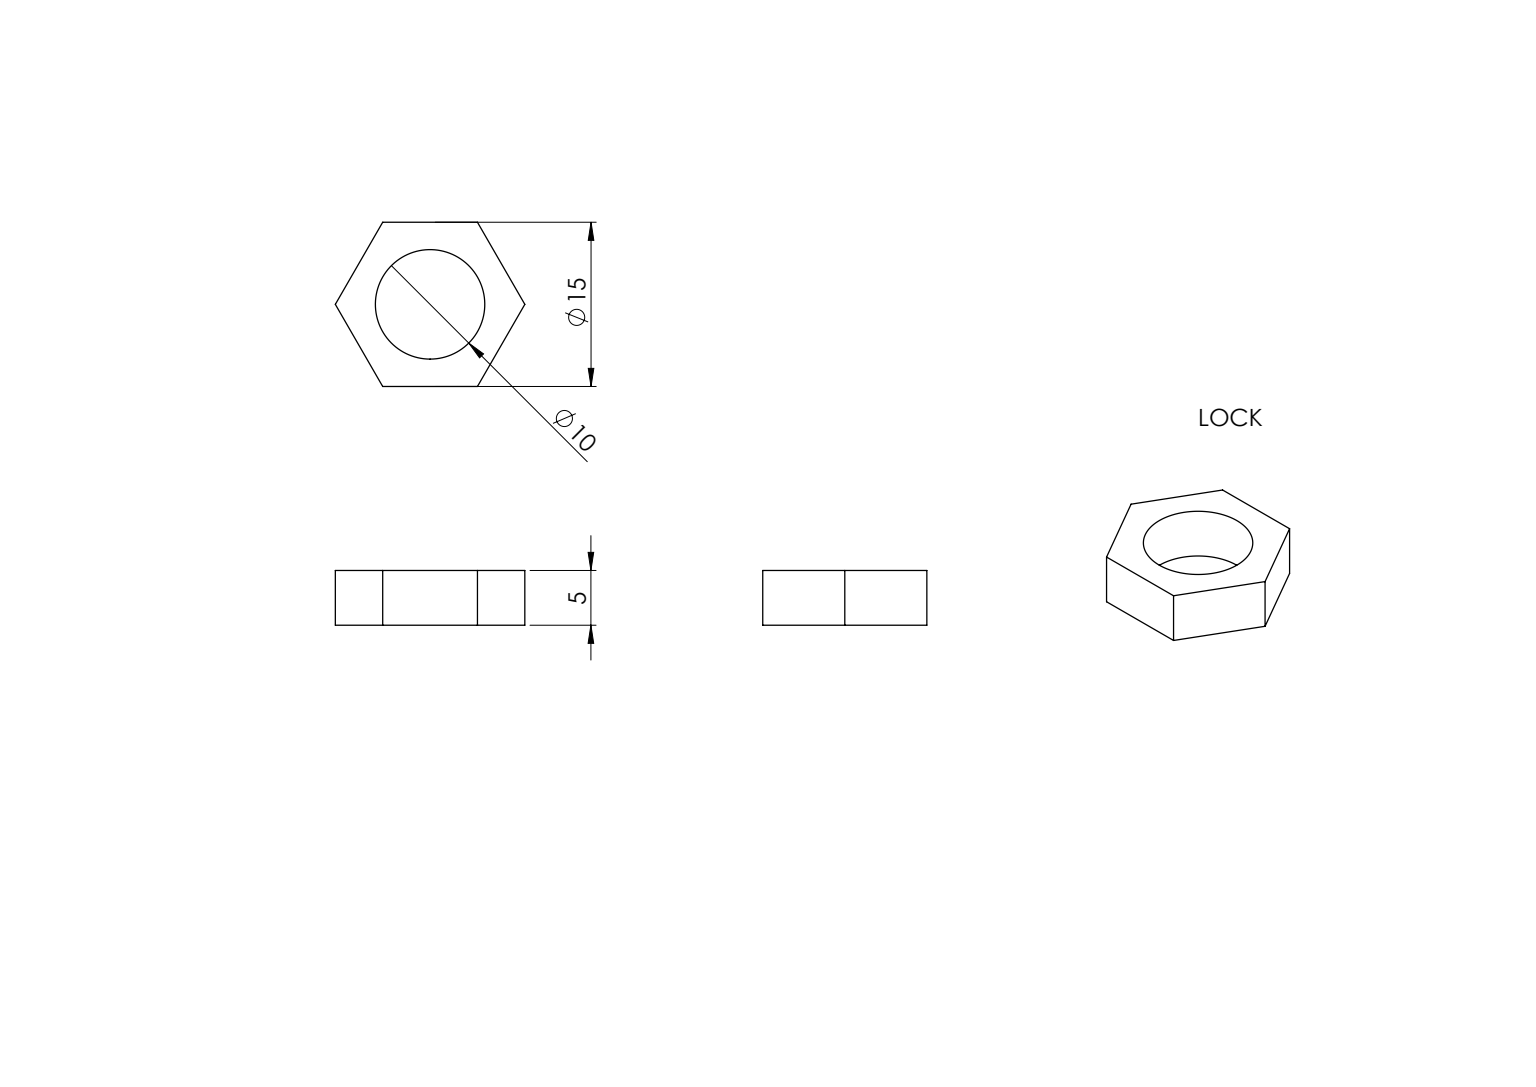
ISO-10303-21;
HEADER;
FILE_DESCRIPTION (('STEP AP214'),
    '1' );
FILE_NAME ('lock.step',
    '2026-10-27T14:18:53',
    ( '' ),
    ( '' ),
    'SwSTEP 2.0',
    'SolidWorks 2026',
    '' );
FILE_SCHEMA (( 'AUTOMOTIVE_DESIGN' ));
ENDSEC;

DATA;
#37=AXIS2_PLACEMENT_3D ( 'NONE', #854, #5957, #5527 ) ;
#40=MECHANICAL_DESIGN_GEOMETRIC_PRESENTATION_REPRESENTATION('',(#808),#5082);
#52=VERTEX_POINT ( 'NONE', #526 ) ;
#68=( NAMED_UNIT ( * ) SI_UNIT ( $, .STERADIAN. ) SOLID_ANGLE_UNIT ( ) );
#112=VECTOR ( 'NONE', #1206, 1000.000000000000000 ) ;
#117=EDGE_LOOP ( 'NONE', ( #4692, #1220, #1894, #1366 ) ) ;
#138=CYLINDRICAL_SURFACE ( 'NONE', #1374, 5.000000000000004441 ) ;
#157=UNCERTAINTY_MEASURE_WITH_UNIT (LENGTH_MEASURE( 1.000000000000000082E-05 ), #285, 'distance_accuracy_value', 'NONE');
#178=CARTESIAN_POINT ( 'NONE',  ( -53.66025403784439618, 45.00000000000000000, 45.00000000000001421 ) ) ;
#187=EDGE_LOOP ( 'NONE', ( #1142, #4922, #3638, #5470 ) ) ;
#212=CARTESIAN_POINT ( 'NONE',  ( -53.66025403784439618, 45.00000000000000000, 45.00000000000001421 ) ) ;
#225=VERTEX_POINT ( 'NONE', #2651 ) ;
#252=CARTESIAN_POINT ( 'NONE',  ( -53.66025403784439618, 40.00000000000000000, 45.00000000000001421 ) ) ;
#278=EDGE_CURVE ( 'NONE', #1461, #3435, #2305, .T. ) ;
#285=( LENGTH_UNIT ( ) NAMED_UNIT ( * ) SI_UNIT ( .MILLI., .METRE. ) );
#298=VECTOR ( 'NONE', #2052, 1000.000000000000227 ) ;
#301=EDGE_CURVE ( 'NONE', #4985, #4357, #4292, .T. ) ;
#309=DIRECTION ( 'NONE',  ( -0.000000000000000000, -1.000000000000000000, -0.000000000000000000 ) ) ;
#322=ORIENTED_EDGE ( 'NONE', *, *, #1089, .F. ) ;
#332=( GEOMETRIC_REPRESENTATION_CONTEXT ( 3 ) GLOBAL_UNCERTAINTY_ASSIGNED_CONTEXT ( ( #1483 ) ) GLOBAL_UNIT_ASSIGNED_CONTEXT ( ( #2789, #1481, #68 ) ) REPRESENTATION_CONTEXT ( 'NONE', 'WORKASPACE' ) );
#335=DIRECTION ( 'NONE',  ( -0.8660254037844390407, 0.000000000000000000, -0.4999999999999993894 ) ) ;
#348=FACE_BOUND ( 'NONE', #3880, .T. ) ;
#364=AXIS2_PLACEMENT_3D ( 'NONE', #2626, #335, #1690 ) ;
#378=CARTESIAN_POINT ( 'NONE',  ( -53.66025403784439618, 45.00000000000000000, 45.00000000000001421 ) ) ;
#394=STYLED_ITEM('',(#6013),#2189);
#396=EDGE_CURVE ( 'NONE', #4357, #4985, #5381, .T. ) ;
#434=CARTESIAN_POINT ( 'NONE',  ( -45.00000000000001421, 40.00000000000000000, 39.99999999999999289 ) ) ;
#465=ORIENTED_EDGE ( 'NONE', *, *, #3725, .F. ) ;
#483=SURFACE_STYLE_USAGE ( .BOTH. , #3752 ) ;
#514=EDGE_LOOP ( 'NONE', ( #4207, #2897 ) ) ;
#526=CARTESIAN_POINT ( 'NONE',  ( -40.66987298107781612, 40.00000000000000000, 37.50000000000000000 ) ) ;
#540=ADVANCED_FACE ( 'NONE', ( #2030 ), #4290, .F. ) ;
#542=VERTEX_POINT ( 'NONE', #968 ) ;
#560=CARTESIAN_POINT ( 'NONE',  ( -40.66987298107781612, 45.00000000000000000, 37.50000000000000000 ) ) ;
#571=( NAMED_UNIT ( * ) SI_UNIT ( $, .STERADIAN. ) SOLID_ANGLE_UNIT ( ) );
#585=ORIENTED_EDGE ( 'NONE', *, *, #2005, .F. ) ;
#588=DIRECTION ( 'NONE',  ( -0.000000000000000000, -1.000000000000000000, -0.000000000000000000 ) ) ;
#593=DIRECTION ( 'NONE',  ( 0.5000000000000004441, 0.000000000000000000, 0.8660254037844383745 ) ) ;
#637=UNCERTAINTY_MEASURE_WITH_UNIT (LENGTH_MEASURE( 1.000000000000000082E-05 ), #2820, 'distance_accuracy_value', 'NONE');
#642=EDGE_CURVE ( 'NONE', #3435, #4780, #1614, .T. ) ;
#643=ADVANCED_FACE ( 'NONE', ( #3491, #4470 ), #669, .F. ) ;
#656=EDGE_CURVE ( 'NONE', #3756, #3717, #1676, .T. ) ;
#667=DIRECTION ( 'NONE',  ( 1.000000000000000000, 0.000000000000000000, 0.000000000000000000 ) ) ;
#669=PLANE ( 'NONE',  #4650 ) ;
#700=PRODUCT_DEFINITION_CONTEXT ( 'detailed design', #4605, 'design' ) ;
#722=DIRECTION ( 'NONE',  ( 0.8660254037844383745, 0.000000000000000000, -0.5000000000000004441 ) ) ;
#754=LINE ( 'NONE', #5791, #1297 ) ;
#798=ORIENTED_EDGE ( 'NONE', *, *, #4836, .F. ) ;
#808=STYLED_ITEM ( 'NONE', ( #3256 ), #3558 ) ;
#820=CARTESIAN_POINT ( 'NONE',  ( -40.66987298107780902, 45.00000000000000000, 52.49999999999999289 ) ) ;
#854=CARTESIAN_POINT ( 'NONE',  ( -45.00000000000001421, 40.00000000000000000, 45.00000000000000000 ) ) ;
#894=DIRECTION ( 'NONE',  ( -0.000000000000000000, -1.000000000000000000, -0.000000000000000000 ) ) ;
#900=VECTOR ( 'NONE', #3820, 1000.000000000000000 ) ;
#909=PRODUCT_DEFINITION_FORMATION_WITH_SPECIFIED_SOURCE ( 'ANY', '', #5230, .NOT_KNOWN. ) ;
#922=ORIENTED_EDGE ( 'NONE', *, *, #1895, .T. ) ;
#968=CARTESIAN_POINT ( 'NONE',  ( -49.33012701892221230, 45.00000000000000000, 37.50000000000000000 ) ) ;
#979=ORIENTED_EDGE ( 'NONE', *, *, #5237, .F. ) ;
#985=DIRECTION ( 'NONE',  ( -0.000000000000000000, -1.000000000000000000, -0.000000000000000000 ) ) ;
#1001=SURFACE_STYLE_FILL_AREA ( #1903 ) ;
#1006=DIRECTION ( 'NONE',  ( 0.000000000000000000, 0.000000000000000000, 1.000000000000000000 ) ) ;
#1034=VERTEX_POINT ( 'NONE', #2118 ) ;
#1037=VERTEX_POINT ( 'NONE', #252 ) ;
#1043=LINE ( 'NONE', #3336, #3266 ) ;
#1059=CARTESIAN_POINT ( 'NONE',  ( -45.00000000000001421, 50.00000000000000000, 45.00000000000000000 ) ) ;
#1067=AXIS2_PLACEMENT_3D ( 'NONE', #3514, #3930, #4365 ) ;
#1076=PLANE ( 'NONE',  #1067 ) ;
#1081=VECTOR ( 'NONE', #2400, 1000.000000000000227 ) ;
#1089=EDGE_CURVE ( 'NONE', #542, #3182, #754, .T. ) ;
#1108=FACE_OUTER_BOUND ( 'NONE', #117, .T. ) ;
#1127=LINE ( 'NONE', #5200, #2704 ) ;
#1142=ORIENTED_EDGE ( 'NONE', *, *, #3725, .T. ) ;
#1183=DIRECTION ( 'NONE',  ( 0.000000000000000000, -0.000000000000000000, 1.000000000000000000 ) ) ;
#1206=DIRECTION ( 'NONE',  ( 1.000000000000000000, 0.000000000000000000, 0.000000000000000000 ) ) ;
#1220=ORIENTED_EDGE ( 'NONE', *, *, #4887, .F. ) ;
#1260=VECTOR ( 'NONE', #1307, 1000.000000000000000 ) ;
#1266=VECTOR ( 'NONE', #1893, 1000.000000000000000 ) ;
#1267=AXIS2_PLACEMENT_3D ( 'NONE', #3330, #3691, #2405 ) ;
#1297=VECTOR ( 'NONE', #2575, 1000.000000000000000 ) ;
#1307=DIRECTION ( 'NONE',  ( -0.4999999999999987232, 0.000000000000000000, 0.8660254037844393737 ) ) ;
#1335=DIRECTION ( 'NONE',  ( 0.5000000000000004441, 0.000000000000000000, 0.8660254037844383745 ) ) ;
#1339=CYLINDRICAL_SURFACE ( 'NONE', #4764, 5.000000000000004441 ) ;
#1365=ORIENTED_EDGE ( 'NONE', *, *, #5237, .T. ) ;
#1366=ORIENTED_EDGE ( 'NONE', *, *, #1089, .T. ) ;
#1374=AXIS2_PLACEMENT_3D ( 'NONE', #1059, #3321, #5173 ) ;
#1411=CARTESIAN_POINT ( 'NONE',  ( -45.00000000000001421, 40.00000000000000000, 50.00000000000000000 ) ) ;
#1428=ORIENTED_EDGE ( 'NONE', *, *, #1448, .T. ) ;
#1432=LINE ( 'NONE', #5620, #2999 ) ;
#1448=EDGE_CURVE ( 'NONE', #1034, #4985, #1043, .T. ) ;
#1461=VERTEX_POINT ( 'NONE', #178 ) ;
#1481=( NAMED_UNIT ( * ) PLANE_ANGLE_UNIT ( ) SI_UNIT ( $, .RADIAN. ) );
#1483=UNCERTAINTY_MEASURE_WITH_UNIT (LENGTH_MEASURE( 1.000000000000000082E-05 ), #2789, 'distance_accuracy_value', 'NONE');
#1500=PRODUCT_DEFINITION_SHAPE ( 'NONE', 'NONE',  #3383 ) ;
#1516=CARTESIAN_POINT ( 'NONE',  ( -40.66987298107781612, 40.00000000000000000, 37.50000000000000000 ) ) ;
#1531=ADVANCED_FACE ( 'NONE', ( #4888 ), #4790, .F. ) ;
#1569=PLANE ( 'NONE',  #4280 ) ;
#1614=LINE ( 'NONE', #3974, #2317 ) ;
#1624=ADVANCED_FACE ( 'NONE', ( #5305 ), #2592, .F. ) ;
#1647=ORIENTED_EDGE ( 'NONE', *, *, #642, .F. ) ;
#1676=LINE ( 'NONE', #2512, #2220 ) ;
#1677=CARTESIAN_POINT ( 'NONE',  ( -49.33012701892221230, 45.00000000000000000, 37.50000000000000000 ) ) ;
#1690=DIRECTION ( 'NONE',  ( -0.4999999999999993339, 0.000000000000000000, 0.8660254037844389297 ) ) ;
#1697=EDGE_LOOP ( 'NONE', ( #2070, #4371, #5360, #922 ) ) ;
#1733=ORIENTED_EDGE ( 'NONE', *, *, #1895, .F. ) ;
#1772=( NAMED_UNIT ( * ) PLANE_ANGLE_UNIT ( ) SI_UNIT ( $, .RADIAN. ) );
#1783=CARTESIAN_POINT ( 'NONE',  ( -49.33012701892221230, 40.00000000000000000, 52.49999999999999289 ) ) ;
#1803=ORIENTED_EDGE ( 'NONE', *, *, #2289, .T. ) ;
#1829=CARTESIAN_POINT ( 'NONE',  ( -49.33012701892221230, 40.00000000000000000, 52.49999999999999289 ) ) ;
#1855=DIRECTION ( 'NONE',  ( -0.000000000000000000, -1.000000000000000000, -0.000000000000000000 ) ) ;
#1862=VECTOR ( 'NONE', #1335, 1000.000000000000000 ) ;
#1878=CLOSED_SHELL ( 'NONE', ( #3533, #1624, #3092, #1531, #3612, #3644, #540, #2608, #643, #4242 ) ) ;
#1890=FACE_OUTER_BOUND ( 'NONE', #1697, .T. ) ;
#1891=AXIS2_PLACEMENT_3D ( 'NONE', #2885, #4258, #5610 ) ;
#1893=DIRECTION ( 'NONE',  ( -0.000000000000000000, -1.000000000000000000, -0.000000000000000000 ) ) ;
#1894=ORIENTED_EDGE ( 'NONE', *, *, #2488, .F. ) ;
#1895=EDGE_CURVE ( 'NONE', #3756, #3278, #1432, .T. ) ;
#1903=FILL_AREA_STYLE ('',( #5191 ) ) ;
#1912=ORIENTED_EDGE ( 'NONE', *, *, #5501, .T. ) ;
#1972=CARTESIAN_POINT ( 'NONE',  ( -40.66987298107780902, 45.00000000000000000, 52.49999999999999289 ) ) ;
#2005=EDGE_CURVE ( 'NONE', #225, #4357, #1127, .T. ) ;
#2013=CARTESIAN_POINT ( 'NONE',  ( -40.66987298107781612, 45.00000000000000000, 37.50000000000000000 ) ) ;
#2024=APPLICATION_CONTEXT ( 'automotive_design' ) ;
#2027=( GEOMETRIC_REPRESENTATION_CONTEXT ( 3 ) GLOBAL_UNCERTAINTY_ASSIGNED_CONTEXT ( ( #157 ) ) GLOBAL_UNIT_ASSIGNED_CONTEXT ( ( #285, #1772, #4074 ) ) REPRESENTATION_CONTEXT ( 'NONE', 'WORKASPACE' ) );
#2030=FACE_OUTER_BOUND ( 'NONE', #2819, .T. ) ;
#2042=CARTESIAN_POINT ( 'NONE',  ( -36.33974596215562514, 40.00000000000000000, 44.99999999999999289 ) ) ;
#2043=CARTESIAN_POINT ( 'NONE',  ( -36.33974596215562514, 45.00000000000000000, 44.99999999999999289 ) ) ;
#2052=DIRECTION ( 'NONE',  ( -0.5000000000000003331, 0.000000000000000000, -0.8660254037844383745 ) ) ;
#2070=ORIENTED_EDGE ( 'NONE', *, *, #2916, .T. ) ;
#2118=CARTESIAN_POINT ( 'NONE',  ( -45.00000000000001421, 45.00000000000000000, 50.00000000000000000 ) ) ;
#2145=AXIS2_PLACEMENT_3D ( 'NONE', #3151, #3509, #5868 ) ;
#2180=EDGE_CURVE ( 'NONE', #3717, #542, #4016, .T. ) ;
#2186=DIRECTION ( 'NONE',  ( 1.000000000000000000, 0.000000000000000000, 0.000000000000000000 ) ) ;
#2189=MANIFOLD_SOLID_BREP ( 'Cavity1', #1878 ) ;
#2220=VECTOR ( 'NONE', #4442, 1000.000000000000227 ) ;
#2235=EDGE_LOOP ( 'NONE', ( #1912, #1733, #2549, #2365 ) ) ;
#2259=VERTEX_POINT ( 'NONE', #2771 ) ;
#2269=DIRECTION ( 'NONE',  ( -0.4999999999999987232, 0.000000000000000000, 0.8660254037844393737 ) ) ;
#2289=EDGE_CURVE ( 'NONE', #225, #1034, #4845, .T. ) ;
#2305=LINE ( 'NONE', #378, #1862 ) ;
#2317=VECTOR ( 'NONE', #2186, 1000.000000000000000 ) ;
#2335=VECTOR ( 'NONE', #5787, 1000.000000000000227 ) ;
#2346=EDGE_CURVE ( 'NONE', #52, #3182, #3347, .T. ) ;
#2365=ORIENTED_EDGE ( 'NONE', *, *, #4397, .T. ) ;
#2392=( NAMED_UNIT ( * ) PLANE_ANGLE_UNIT ( ) SI_UNIT ( $, .RADIAN. ) );
#2400=DIRECTION ( 'NONE',  ( 0.4999999999999993894, 0.000000000000000000, -0.8660254037844389297 ) ) ;
#2404=EDGE_LOOP ( 'NONE', ( #4237, #322, #5705, #2478 ) ) ;
#2405=DIRECTION ( 'NONE',  ( 0.5000000000000003331, 0.000000000000000000, 0.8660254037844383745 ) ) ;
#2419=ORIENTED_EDGE ( 'NONE', *, *, #4247, .T. ) ;
#2434=ORIENTED_EDGE ( 'NONE', *, *, #2346, .F. ) ;
#2441=PLANE ( 'NONE',  #1267 ) ;
#2478=ORIENTED_EDGE ( 'NONE', *, *, #4898, .T. ) ;
#2488=EDGE_CURVE ( 'NONE', #542, #1461, #3977, .T. ) ;
#2512=CARTESIAN_POINT ( 'NONE',  ( -36.33974596215562514, 45.00000000000000000, 44.99999999999999289 ) ) ;
#2549=ORIENTED_EDGE ( 'NONE', *, *, #4247, .F. ) ;
#2564=SHAPE_DEFINITION_REPRESENTATION ( #1500, #2622 ) ;
#2575=DIRECTION ( 'NONE',  ( -0.000000000000000000, -1.000000000000000000, -0.000000000000000000 ) ) ;
#2581=DIRECTION ( 'NONE',  ( 0.000000000000000000, 1.000000000000000000, 0.000000000000000000 ) ) ;
#2592=PLANE ( 'NONE',  #364 ) ;
#2608=ADVANCED_FACE ( 'NONE', ( #348, #3139 ), #4037, .T. ) ;
#2622=SHAPE_REPRESENTATION ( 'lock', ( #5080 ), #332 ) ;
#2626=CARTESIAN_POINT ( 'NONE',  ( -40.66987298107780902, 45.00000000000000000, 52.49999999999999289 ) ) ;
#2651=CARTESIAN_POINT ( 'NONE',  ( -45.00000000000001421, 45.00000000000000000, 39.99999999999999289 ) ) ;
#2655=ORIENTED_EDGE ( 'NONE', *, *, #5921, .T. ) ;
#2676=AXIS2_PLACEMENT_3D ( 'NONE', #2013, #5366, #4398 ) ;
#2704=VECTOR ( 'NONE', #588, 1000.000000000000000 ) ;
#2750=DIRECTION ( 'NONE',  ( 0.000000000000000000, 0.000000000000000000, -1.000000000000000000 ) ) ;
#2771=CARTESIAN_POINT ( 'NONE',  ( -40.66987298107780902, 40.00000000000000000, 52.49999999999999289 ) ) ;
#2789=( LENGTH_UNIT ( ) NAMED_UNIT ( * ) SI_UNIT ( .MILLI., .METRE. ) );
#2812=ORIENTED_EDGE ( 'NONE', *, *, #301, .T. ) ;
#2819=EDGE_LOOP ( 'NONE', ( #3590, #5383, #1647, #2655 ) ) ;
#2820=( LENGTH_UNIT ( ) NAMED_UNIT ( * ) SI_UNIT ( .MILLI., .METRE. ) );
#2824=ORIENTED_EDGE ( 'NONE', *, *, #5501, .F. ) ;
#2877=ORIENTED_EDGE ( 'NONE', *, *, #2978, .F. ) ;
#2878=SHAPE_REPRESENTATION_RELATIONSHIP ( 'NONE' , 'NONE' ,  #2622, #3558 ) ;
#2885=CARTESIAN_POINT ( 'NONE',  ( -45.00000000000001421, 40.00000000000000000, 45.00000000000000000 ) ) ;
#2897=ORIENTED_EDGE ( 'NONE', *, *, #301, .F. ) ;
#2916=EDGE_CURVE ( 'NONE', #3278, #52, #2939, .T. ) ;
#2921=LINE ( 'NONE', #1972, #1081 ) ;
#2939=LINE ( 'NONE', #3871, #298 ) ;
#2975=ORIENTED_EDGE ( 'NONE', *, *, #396, .T. ) ;
#2978=EDGE_CURVE ( 'NONE', #3182, #1037, #3121, .T. ) ;
#2999=VECTOR ( 'NONE', #985, 1000.000000000000000 ) ;
#3010=VECTOR ( 'NONE', #2269, 1000.000000000000000 ) ;
#3015=VECTOR ( 'NONE', #3271, 1000.000000000000000 ) ;
#3026=PRODUCT_CONTEXT ( 'NONE', #2024, 'mechanical' ) ;
#3036=ORIENTED_EDGE ( 'NONE', *, *, #278, .T. ) ;
#3050=DIRECTION ( 'NONE',  ( -1.000000000000000000, 0.000000000000000000, 0.000000000000000000 ) ) ;
#3060=CARTESIAN_POINT ( 'NONE',  ( -40.66987298107781612, 45.00000000000000000, 37.50000000000000000 ) ) ;
#3064=EDGE_LOOP ( 'NONE', ( #3201, #4812, #4033, #2975 ) ) ;
#3092=ADVANCED_FACE ( 'NONE', ( #1890 ), #2441, .F. ) ;
#3100=VECTOR ( 'NONE', #3795, 1000.000000000000000 ) ;
#3121=LINE ( 'NONE', #3217, #3010 ) ;
#3139=FACE_OUTER_BOUND ( 'NONE', #4475, .T. ) ;
#3151=CARTESIAN_POINT ( 'NONE',  ( -45.00000000000001421, 45.00000000000000000, 45.00000000000000000 ) ) ;
#3171=AXIS2_PLACEMENT_3D ( 'NONE', #5672, #3372, #5138 ) ;
#3182=VERTEX_POINT ( 'NONE', #3269 ) ;
#3201=ORIENTED_EDGE ( 'NONE', *, *, #1448, .F. ) ;
#3217=CARTESIAN_POINT ( 'NONE',  ( -49.33012701892221230, 40.00000000000000000, 37.50000000000000000 ) ) ;
#3256=PRESENTATION_STYLE_ASSIGNMENT (( #483 ) ) ;
#3266=VECTOR ( 'NONE', #4307, 1000.000000000000000 ) ;
#3269=CARTESIAN_POINT ( 'NONE',  ( -49.33012701892221230, 40.00000000000000000, 37.50000000000000000 ) ) ;
#3271=DIRECTION ( 'NONE',  ( -0.000000000000000000, -1.000000000000000000, -0.000000000000000000 ) ) ;
#3278=VERTEX_POINT ( 'NONE', #2042 ) ;
#3309=CIRCLE ( 'NONE', #2145, 5.000000000000004441 ) ;
#3321=DIRECTION ( 'NONE',  ( -0.000000000000000000, -1.000000000000000000, -0.000000000000000000 ) ) ;
#3330=CARTESIAN_POINT ( 'NONE',  ( -36.33974596215562514, 45.00000000000000000, 44.99999999999999289 ) ) ;
#3336=CARTESIAN_POINT ( 'NONE',  ( -45.00000000000001421, 50.00000000000000000, 50.00000000000000000 ) ) ;
#3347=LINE ( 'NONE', #1516, #3100 ) ;
#3372=DIRECTION ( 'NONE',  ( 0.000000000000000000, 0.000000000000000000, -1.000000000000000000 ) ) ;
#3383=PRODUCT_DEFINITION ( 'UNKNOWN', '', #909, #700 ) ;
#3435=VERTEX_POINT ( 'NONE', #4971 ) ;
#3482=VECTOR ( 'NONE', #3050, 1000.000000000000000 ) ;
#3491=FACE_BOUND ( 'NONE', #514, .T. ) ;
#3509=DIRECTION ( 'NONE',  ( -0.000000000000000000, -1.000000000000000000, -0.000000000000000000 ) ) ;
#3514=CARTESIAN_POINT ( 'NONE',  ( -49.33012701892221230, 45.00000000000000000, 37.50000000000000000 ) ) ;
#3523=COLOUR_RGB ( '',0.8941176470588234615, 0.8941176470588234615, 0.8941176470588234615 ) ;
#3527=CARTESIAN_POINT ( 'NONE',  ( 0.000000000000000000, 0.000000000000000000, 0.000000000000000000 ) ) ;
#3533=ADVANCED_FACE ( 'NONE', ( #5505 ), #1339, .F. ) ;
#3558=ADVANCED_BREP_SHAPE_REPRESENTATION ( '', ( #2189, #5080 ), #332 ) ;
#3583=DIRECTION ( 'NONE',  ( 0.000000000000000000, -0.000000000000000000, 1.000000000000000000 ) ) ;
#3590=ORIENTED_EDGE ( 'NONE', *, *, #4836, .T. ) ;
#3612=ADVANCED_FACE ( 'NONE', ( #1108 ), #1076, .F. ) ;
#3625=CARTESIAN_POINT ( 'NONE',  ( -40.66987298107781612, 45.00000000000000000, 37.50000000000000000 ) ) ;
#3638=ORIENTED_EDGE ( 'NONE', *, *, #278, .F. ) ;
#3644=ADVANCED_FACE ( 'NONE', ( #5720 ), #1569, .F. ) ;
#3691=DIRECTION ( 'NONE',  ( -0.8660254037844384856, 0.000000000000000000, 0.5000000000000004441 ) ) ;
#3717=VERTEX_POINT ( 'NONE', #3060 ) ;
#3725=EDGE_CURVE ( 'NONE', #1037, #4171, #4820, .T. ) ;
#3752=SURFACE_SIDE_STYLE ('',( #1001 ) ) ;
#3756=VERTEX_POINT ( 'NONE', #2043 ) ;
#3771=CARTESIAN_POINT ( 'NONE',  ( -53.66025403784439618, 45.00000000000000000, 45.00000000000001421 ) ) ;
#3795=DIRECTION ( 'NONE',  ( -1.000000000000000000, 0.000000000000000000, 0.000000000000000000 ) ) ;
#3820=DIRECTION ( 'NONE',  ( -0.000000000000000000, -1.000000000000000000, -0.000000000000000000 ) ) ;
#3871=CARTESIAN_POINT ( 'NONE',  ( -36.33974596215562514, 40.00000000000000000, 44.99999999999999289 ) ) ;
#3880=EDGE_LOOP ( 'NONE', ( #1803, #1365 ) ) ;
#3930=DIRECTION ( 'NONE',  ( 0.8660254037844393737, -0.000000000000000000, 0.4999999999999987232 ) ) ;
#3974=CARTESIAN_POINT ( 'NONE',  ( -49.33012701892221230, 45.00000000000000000, 52.49999999999999289 ) ) ;
#3977=LINE ( 'NONE', #1677, #1260 ) ;
#4016=LINE ( 'NONE', #3625, #3482 ) ;
#4033=ORIENTED_EDGE ( 'NONE', *, *, #2005, .T. ) ;
#4036=DIRECTION ( 'NONE',  ( 0.000000000000000000, 1.000000000000000000, 0.000000000000000000 ) ) ;
#4037=PLANE ( 'NONE',  #4563 ) ;
#4063=AXIS2_PLACEMENT_3D ( 'NONE', #5614, #1855, #1006 ) ;
#4074=( NAMED_UNIT ( * ) SI_UNIT ( $, .STERADIAN. ) SOLID_ANGLE_UNIT ( ) );
#4171=VERTEX_POINT ( 'NONE', #1829 ) ;
#4207=ORIENTED_EDGE ( 'NONE', *, *, #396, .F. ) ;
#4237=ORIENTED_EDGE ( 'NONE', *, *, #2346, .T. ) ;
#4242=ADVANCED_FACE ( 'NONE', ( #5221 ), #138, .F. ) ;
#4247=EDGE_CURVE ( 'NONE', #4780, #3756, #2921, .T. ) ;
#4255=ORIENTED_EDGE ( 'NONE', *, *, #656, .T. ) ;
#4258=DIRECTION ( 'NONE',  ( -0.000000000000000000, -1.000000000000000000, -0.000000000000000000 ) ) ;
#4280=AXIS2_PLACEMENT_3D ( 'NONE', #212, #722, #5785 ) ;
#4290=PLANE ( 'NONE',  #3171 ) ;
#4292=CIRCLE ( 'NONE', #37, 5.000000000000004441 ) ;
#4307=DIRECTION ( 'NONE',  ( -0.000000000000000000, -1.000000000000000000, -0.000000000000000000 ) ) ;
#4357=VERTEX_POINT ( 'NONE', #434 ) ;
#4365=DIRECTION ( 'NONE',  ( 0.4999999999999987232, 0.000000000000000000, -0.8660254037844393737 ) ) ;
#4371=ORIENTED_EDGE ( 'NONE', *, *, #4898, .F. ) ;
#4397=EDGE_CURVE ( 'NONE', #4780, #2259, #5521, .T. ) ;
#4398=DIRECTION ( 'NONE',  ( 1.000000000000000000, 0.000000000000000000, -0.000000000000000000 ) ) ;
#4442=DIRECTION ( 'NONE',  ( -0.5000000000000003331, 0.000000000000000000, -0.8660254037844383745 ) ) ;
#4470=FACE_OUTER_BOUND ( 'NONE', #5617, .T. ) ;
#4475=EDGE_LOOP ( 'NONE', ( #2419, #4255, #5288, #5888, #3036, #4745 ) ) ;
#4497=LINE ( 'NONE', #1783, #112 ) ;
#4563=AXIS2_PLACEMENT_3D ( 'NONE', #5886, #2581, #3583 ) ;
#4605=APPLICATION_CONTEXT ( 'automotive_design' ) ;
#4647=MECHANICAL_DESIGN_GEOMETRIC_PRESENTATION_REPRESENTATION('',(#394),#2027);
#4650=AXIS2_PLACEMENT_3D ( 'NONE', #4901, #4036, #1183 ) ;
#4686=CARTESIAN_POINT ( 'NONE',  ( -49.33012701892221230, 45.00000000000000000, 52.49999999999999289 ) ) ;
#4692=ORIENTED_EDGE ( 'NONE', *, *, #2978, .T. ) ;
#4745=ORIENTED_EDGE ( 'NONE', *, *, #642, .T. ) ;
#4764=AXIS2_PLACEMENT_3D ( 'NONE', #5062, #894, #2750 ) ;
#4773=LINE ( 'NONE', #4686, #900 ) ;
#4780=VERTEX_POINT ( 'NONE', #5014 ) ;
#4790=PLANE ( 'NONE',  #2676 ) ;
#4812=ORIENTED_EDGE ( 'NONE', *, *, #2289, .F. ) ;
#4820=LINE ( 'NONE', #5279, #5727 ) ;
#4831=DIRECTION ( 'NONE',  ( 0.000000000000000000, 0.000000000000000000, 1.000000000000000000 ) ) ;
#4836=EDGE_CURVE ( 'NONE', #4171, #2259, #4497, .T. ) ;
#4845=CIRCLE ( 'NONE', #4063, 5.000000000000004441 ) ;
#4853=CARTESIAN_POINT ( 'NONE',  ( -40.66987298107780902, 40.00000000000000000, 52.49999999999999289 ) ) ;
#4887=EDGE_CURVE ( 'NONE', #1461, #1037, #5124, .T. ) ;
#4888=FACE_OUTER_BOUND ( 'NONE', #2404, .T. ) ;
#4898=EDGE_CURVE ( 'NONE', #3717, #52, #5156, .T. ) ;
#4901=CARTESIAN_POINT ( 'NONE',  ( 0.000000000000000000, 40.00000000000000000, 0.000000000000000000 ) ) ;
#4922=ORIENTED_EDGE ( 'NONE', *, *, #5921, .F. ) ;
#4971=CARTESIAN_POINT ( 'NONE',  ( -49.33012701892221230, 45.00000000000000000, 52.49999999999999289 ) ) ;
#4985=VERTEX_POINT ( 'NONE', #1411 ) ;
#5014=CARTESIAN_POINT ( 'NONE',  ( -40.66987298107780902, 45.00000000000000000, 52.49999999999999289 ) ) ;
#5062=CARTESIAN_POINT ( 'NONE',  ( -45.00000000000001421, 50.00000000000000000, 45.00000000000000000 ) ) ;
#5080=AXIS2_PLACEMENT_3D ( 'NONE', #3527, #4831, #667 ) ;
#5082=( GEOMETRIC_REPRESENTATION_CONTEXT ( 3 ) GLOBAL_UNCERTAINTY_ASSIGNED_CONTEXT ( ( #637 ) ) GLOBAL_UNIT_ASSIGNED_CONTEXT ( ( #2820, #2392, #571 ) ) REPRESENTATION_CONTEXT ( 'NONE', 'WORKASPACE' ) );
#5124=LINE ( 'NONE', #3771, #3015 ) ;
#5138=DIRECTION ( 'NONE',  ( -1.000000000000000000, 0.000000000000000000, -0.000000000000000000 ) ) ;
#5156=LINE ( 'NONE', #560, #1266 ) ;
#5173=DIRECTION ( 'NONE',  ( 0.000000000000000000, 0.000000000000000000, -1.000000000000000000 ) ) ;
#5190=EDGE_LOOP ( 'NONE', ( #979, #1428, #2812, #585 ) ) ;
#5191=FILL_AREA_STYLE_COLOUR ( '', #3523 ) ;
#5200=CARTESIAN_POINT ( 'NONE',  ( -45.00000000000001421, 50.00000000000000000, 39.99999999999999289 ) ) ;
#5221=FACE_OUTER_BOUND ( 'NONE', #3064, .T. ) ;
#5230=PRODUCT ( 'lock', 'lock', '', ( #3026 ) ) ;
#5237=EDGE_CURVE ( 'NONE', #1034, #225, #3309, .T. ) ;
#5279=CARTESIAN_POINT ( 'NONE',  ( -53.66025403784439618, 40.00000000000000000, 45.00000000000001421 ) ) ;
#5288=ORIENTED_EDGE ( 'NONE', *, *, #2180, .T. ) ;
#5305=FACE_OUTER_BOUND ( 'NONE', #2235, .T. ) ;
#5308=LINE ( 'NONE', #4853, #2335 ) ;
#5360=ORIENTED_EDGE ( 'NONE', *, *, #656, .F. ) ;
#5366=DIRECTION ( 'NONE',  ( 0.000000000000000000, -0.000000000000000000, 1.000000000000000000 ) ) ;
#5381=CIRCLE ( 'NONE', #1891, 5.000000000000004441 ) ;
#5383=ORIENTED_EDGE ( 'NONE', *, *, #4397, .F. ) ;
#5452=VECTOR ( 'NONE', #309, 1000.000000000000000 ) ;
#5470=ORIENTED_EDGE ( 'NONE', *, *, #4887, .T. ) ;
#5501=EDGE_CURVE ( 'NONE', #2259, #3278, #5308, .T. ) ;
#5505=FACE_OUTER_BOUND ( 'NONE', #5190, .T. ) ;
#5521=LINE ( 'NONE', #820, #5452 ) ;
#5527=DIRECTION ( 'NONE',  ( 0.000000000000000000, 0.000000000000000000, 1.000000000000000000 ) ) ;
#5610=DIRECTION ( 'NONE',  ( 0.000000000000000000, 0.000000000000000000, 1.000000000000000000 ) ) ;
#5614=CARTESIAN_POINT ( 'NONE',  ( -45.00000000000001421, 45.00000000000000000, 45.00000000000000000 ) ) ;
#5617=EDGE_LOOP ( 'NONE', ( #2824, #798, #465, #2877, #2434, #5665 ) ) ;
#5620=CARTESIAN_POINT ( 'NONE',  ( -36.33974596215562514, 45.00000000000000000, 44.99999999999999289 ) ) ;
#5665=ORIENTED_EDGE ( 'NONE', *, *, #2916, .F. ) ;
#5672=CARTESIAN_POINT ( 'NONE',  ( -49.33012701892221230, 45.00000000000000000, 52.49999999999999289 ) ) ;
#5705=ORIENTED_EDGE ( 'NONE', *, *, #2180, .F. ) ;
#5720=FACE_OUTER_BOUND ( 'NONE', #187, .T. ) ;
#5727=VECTOR ( 'NONE', #593, 1000.000000000000000 ) ;
#5785=DIRECTION ( 'NONE',  ( -0.5000000000000004441, 0.000000000000000000, -0.8660254037844383745 ) ) ;
#5787=DIRECTION ( 'NONE',  ( 0.4999999999999993894, 0.000000000000000000, -0.8660254037844389297 ) ) ;
#5791=CARTESIAN_POINT ( 'NONE',  ( -49.33012701892221230, 45.00000000000000000, 37.50000000000000000 ) ) ;
#5868=DIRECTION ( 'NONE',  ( 0.000000000000000000, 0.000000000000000000, 1.000000000000000000 ) ) ;
#5886=CARTESIAN_POINT ( 'NONE',  ( 0.000000000000000000, 45.00000000000000000, 0.000000000000000000 ) ) ;
#5888=ORIENTED_EDGE ( 'NONE', *, *, #2488, .T. ) ;
#5921=EDGE_CURVE ( 'NONE', #3435, #4171, #4773, .T. ) ;
#5957=DIRECTION ( 'NONE',  ( -0.000000000000000000, -1.000000000000000000, -0.000000000000000000 ) ) ;
#6007=COLOUR_RGB('Sky Blue',0.24,0.69,0.87);
#6008=FILL_AREA_STYLE_COLOUR('',#6007);
#6009=FILL_AREA_STYLE('',(#6008));
#6010=SURFACE_STYLE_FILL_AREA(#6009);
#6011=SURFACE_SIDE_STYLE('',(#6010));
#6012=SURFACE_STYLE_USAGE(.BOTH.,#6011);
#6013=PRESENTATION_STYLE_ASSIGNMENT((#6012));
ENDSEC;
END-ISO-10303-21;
